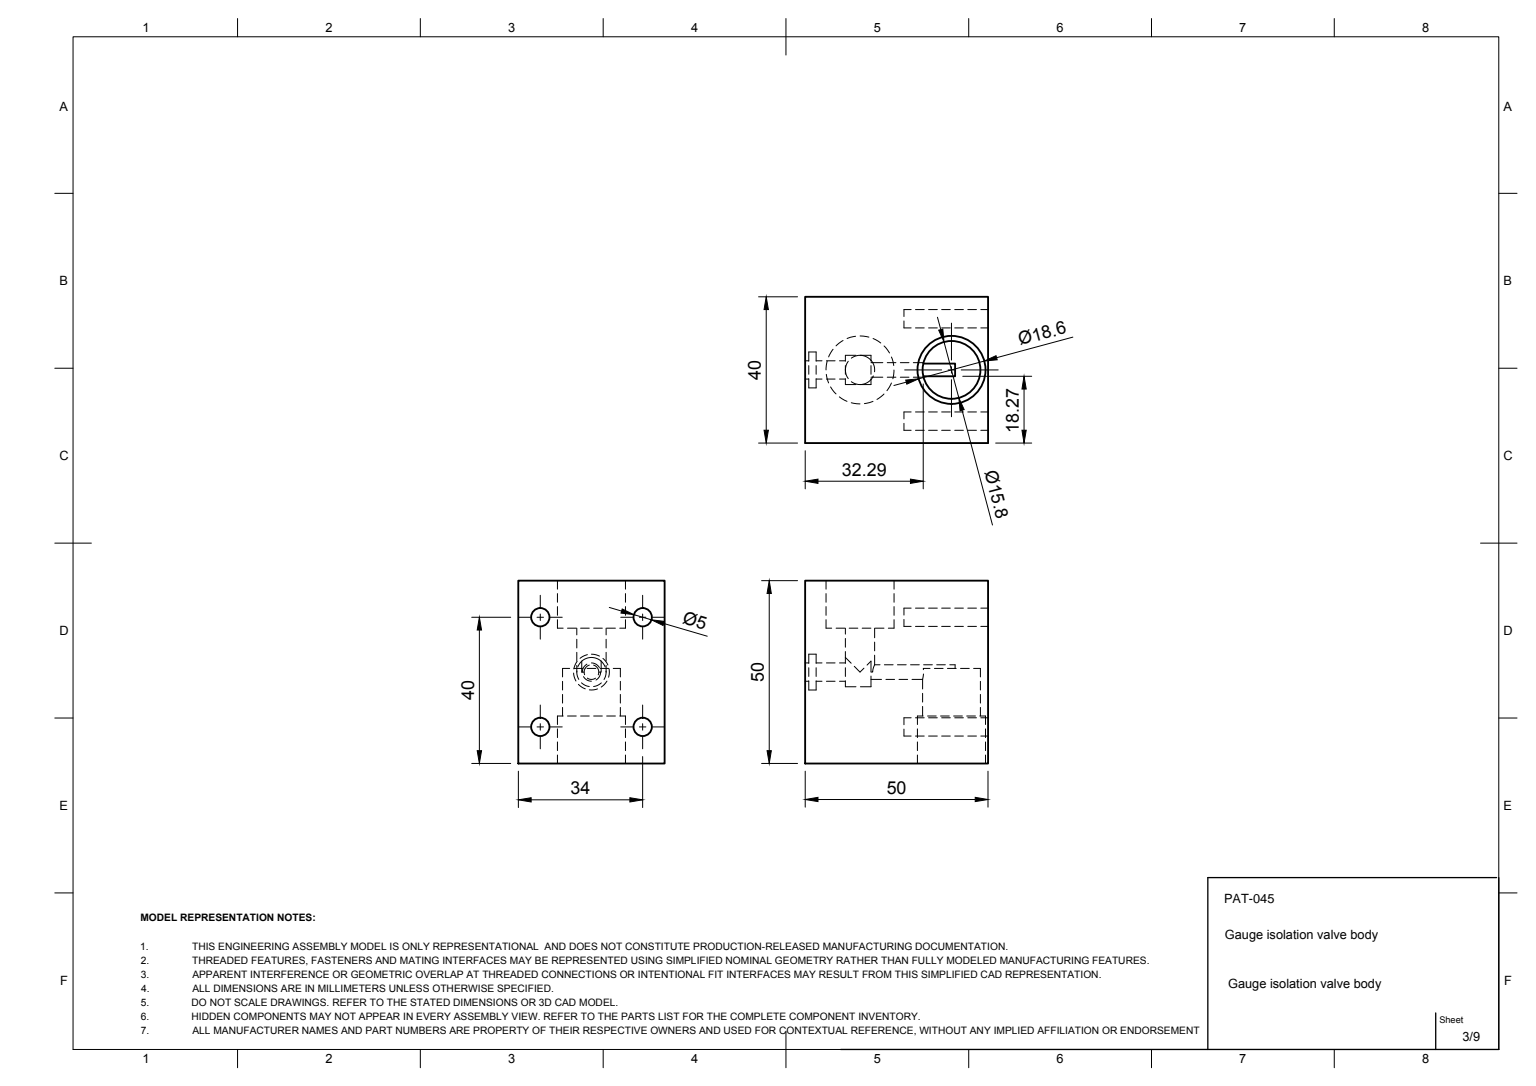
ISO-10303-21;
HEADER;
/* Generated by software containing ST-Developer
 * from STEP Tools, Inc. (www.steptools.com) 
 */

FILE_DESCRIPTION(
/* description */ ('Gauge isolation and snubber set'),
/* implementation_level */ '2;1');

FILE_NAME(
/* name */ 'Gauge isolation valve body.step',
/* time_stamp */ '2026-10-29T16:58:15-07:00',
/* author */ (''),
/* organization */ (''),
/* preprocessor_version */ 'ST-DEVELOPER v20.2',
/* originating_system */ 'Autodesk Translation Framework v15.17.0.0',
/* authorisation */ '');

FILE_SCHEMA (('AUTOMOTIVE_DESIGN { 1 0 10303 214 3 1 1 }'));
ENDSEC;

DATA;
#10=MECHANICAL_DESIGN_GEOMETRIC_PRESENTATION_REPRESENTATION('',(#92),#4043);
#76=SHAPE_REPRESENTATION_RELATIONSHIP('SRR','None',#4083,#84);
#84=ADVANCED_BREP_SHAPE_REPRESENTATION('',(#102),#4035);
#92=STYLED_ITEM('',(#4176),#102);
#102=MANIFOLD_SOLID_BREP('Body1',#2209);
#112=FACE_BOUND('',#379,.T.);
#113=FACE_BOUND('',#382,.T.);
#114=FACE_BOUND('',#384,.T.);
#115=FACE_BOUND('',#389,.T.);
#116=FACE_BOUND('',#397,.T.);
#117=FACE_BOUND('',#400,.T.);
#118=FACE_BOUND('',#403,.T.);
#119=FACE_BOUND('',#405,.T.);
#120=FACE_BOUND('',#407,.T.);
#121=FACE_BOUND('',#408,.T.);
#122=FACE_BOUND('',#409,.T.);
#123=FACE_BOUND('',#410,.T.);
#153=B_SPLINE_CURVE_WITH_KNOTS('',3,(#3286,#3287,#3288,#3289,#3290,#3291,
#3292,#3293,#3294,#3295,#3296,#3297,#3298,#3299,#3300,#3301,#3302,#3303),
 .UNSPECIFIED.,.F.,.F.,(4,2,2,2,2,2,2,2,4),(0.,0.0769830401762947,0.153966080352589,
0.230739261017803,0.307512441683016,0.384285622348229,0.461058803013443,
0.538041843189737,0.615024883366032),.UNSPECIFIED.);
#154=B_SPLINE_CURVE_WITH_KNOTS('',3,(#3360,#3361,#3362,#3363,#3364,#3365,
#3366,#3367,#3368,#3369,#3370,#3371,#3372,#3373,#3374),.UNSPECIFIED.,.F.,
 .F.,(4,2,2,2,3,2,4),(-0.302773934408822,-0.227086024595877,-0.151398114782933,
-0.0756990573914662,0.,0.0756990573914663,0.1003787904191),
 .UNSPECIFIED.);
#155=B_SPLINE_CURVE_WITH_KNOTS('',3,(#3377,#3378,#3379,#3380,#3381,#3382,
#3383,#3384,#3385,#3386,#3387,#3388,#3389,#3390),.UNSPECIFIED.,.F.,.F.,
(4,2,2,2,2,2,4),(-0.705926659236745,-0.681246926209111,-0.605547868817645,
-0.529848811426178,-0.454149754034712,-0.378461844221767,-0.302773934408822),
 .UNSPECIFIED.);
#164=PLANE('',#2319);
#165=PLANE('',#2323);
#166=PLANE('',#2327);
#167=PLANE('',#2331);
#168=PLANE('',#2332);
#169=PLANE('',#2339);
#170=PLANE('',#2343);
#171=PLANE('',#2347);
#172=PLANE('',#2349);
#173=PLANE('',#2358);
#174=PLANE('',#2359);
#175=PLANE('',#2362);
#176=PLANE('',#2365);
#177=PLANE('',#2372);
#178=PLANE('',#2373);
#179=PLANE('',#2374);
#180=PLANE('',#2375);
#181=PLANE('',#2376);
#182=PLANE('',#2377);
#183=PLANE('',#2378);
#241=FACE_OUTER_BOUND('',#365,.T.);
#242=FACE_OUTER_BOUND('',#366,.T.);
#243=FACE_OUTER_BOUND('',#367,.T.);
#244=FACE_OUTER_BOUND('',#368,.T.);
#245=FACE_OUTER_BOUND('',#369,.T.);
#246=FACE_OUTER_BOUND('',#370,.T.);
#247=FACE_OUTER_BOUND('',#371,.T.);
#248=FACE_OUTER_BOUND('',#372,.T.);
#249=FACE_OUTER_BOUND('',#373,.T.);
#250=FACE_OUTER_BOUND('',#374,.T.);
#251=FACE_OUTER_BOUND('',#375,.T.);
#252=FACE_OUTER_BOUND('',#376,.T.);
#253=FACE_OUTER_BOUND('',#377,.T.);
#254=FACE_OUTER_BOUND('',#378,.T.);
#255=FACE_OUTER_BOUND('',#380,.T.);
#256=FACE_OUTER_BOUND('',#381,.T.);
#257=FACE_OUTER_BOUND('',#383,.T.);
#258=FACE_OUTER_BOUND('',#385,.T.);
#259=FACE_OUTER_BOUND('',#386,.T.);
#260=FACE_OUTER_BOUND('',#387,.T.);
#261=FACE_OUTER_BOUND('',#388,.T.);
#262=FACE_OUTER_BOUND('',#390,.T.);
#263=FACE_OUTER_BOUND('',#391,.T.);
#264=FACE_OUTER_BOUND('',#392,.T.);
#265=FACE_OUTER_BOUND('',#393,.T.);
#266=FACE_OUTER_BOUND('',#394,.T.);
#267=FACE_OUTER_BOUND('',#395,.T.);
#268=FACE_OUTER_BOUND('',#396,.T.);
#269=FACE_OUTER_BOUND('',#398,.T.);
#270=FACE_OUTER_BOUND('',#399,.T.);
#271=FACE_OUTER_BOUND('',#401,.T.);
#272=FACE_OUTER_BOUND('',#402,.T.);
#273=FACE_OUTER_BOUND('',#404,.T.);
#274=FACE_OUTER_BOUND('',#406,.T.);
#365=EDGE_LOOP('',(#1461,#1462,#1463,#1464,#1465));
#366=EDGE_LOOP('',(#1466,#1467,#1468,#1469));
#367=EDGE_LOOP('',(#1470));
#368=EDGE_LOOP('',(#1471,#1472,#1473,#1474));
#369=EDGE_LOOP('',(#1475));
#370=EDGE_LOOP('',(#1476,#1477,#1478,#1479));
#371=EDGE_LOOP('',(#1480));
#372=EDGE_LOOP('',(#1481,#1482,#1483,#1484));
#373=EDGE_LOOP('',(#1485));
#374=EDGE_LOOP('',(#1486,#1487,#1488));
#375=EDGE_LOOP('',(#1489,#1490,#1491,#1492,#1493,#1494,#1495,#1496,#1497,
#1498,#1499,#1500));
#376=EDGE_LOOP('',(#1501,#1502,#1503));
#377=EDGE_LOOP('',(#1504,#1505,#1506,#1507));
#378=EDGE_LOOP('',(#1508));
#379=EDGE_LOOP('',(#1509));
#380=EDGE_LOOP('',(#1510,#1511,#1512,#1513));
#381=EDGE_LOOP('',(#1514));
#382=EDGE_LOOP('',(#1515));
#383=EDGE_LOOP('',(#1516));
#384=EDGE_LOOP('',(#1517));
#385=EDGE_LOOP('',(#1518,#1519,#1520,#1521));
#386=EDGE_LOOP('',(#1522,#1523,#1524,#1525));
#387=EDGE_LOOP('',(#1526,#1527,#1528,#1529,#1530));
#388=EDGE_LOOP('',(#1531,#1532));
#389=EDGE_LOOP('',(#1533));
#390=EDGE_LOOP('',(#1534,#1535,#1536,#1537,#1538,#1539,#1540,#1541));
#391=EDGE_LOOP('',(#1542,#1543));
#392=EDGE_LOOP('',(#1544,#1545,#1546,#1547,#1548,#1549,#1550,#1551,#1552,
#1553,#1554,#1555));
#393=EDGE_LOOP('',(#1556,#1557,#1558,#1559));
#394=EDGE_LOOP('',(#1560,#1561,#1562,#1563,#1564,#1565));
#395=EDGE_LOOP('',(#1566,#1567,#1568,#1569));
#396=EDGE_LOOP('',(#1570));
#397=EDGE_LOOP('',(#1571));
#398=EDGE_LOOP('',(#1572,#1573,#1574,#1575));
#399=EDGE_LOOP('',(#1576,#1577,#1578,#1579));
#400=EDGE_LOOP('',(#1580));
#401=EDGE_LOOP('',(#1581,#1582,#1583,#1584));
#402=EDGE_LOOP('',(#1585,#1586,#1587,#1588));
#403=EDGE_LOOP('',(#1589));
#404=EDGE_LOOP('',(#1590,#1591,#1592,#1593));
#405=EDGE_LOOP('',(#1594));
#406=EDGE_LOOP('',(#1595,#1596,#1597,#1598));
#407=EDGE_LOOP('',(#1599));
#408=EDGE_LOOP('',(#1600));
#409=EDGE_LOOP('',(#1601));
#410=EDGE_LOOP('',(#1602));
#530=ELLIPSE('',#2313,0.565685424949238,0.4);
#531=ELLIPSE('',#2314,0.565685424949238,0.4);
#532=ELLIPSE('',#2336,0.565685424949238,0.4);
#533=ELLIPSE('',#2337,0.565685424949238,0.4);
#534=CIRCLE('',#2312,0.4);
#535=CIRCLE('',#2315,0.4);
#536=CIRCLE('',#2317,0.25);
#537=CIRCLE('',#2318,0.25);
#538=CIRCLE('',#2321,0.25);
#539=CIRCLE('',#2322,0.25);
#540=CIRCLE('',#2325,0.25);
#541=CIRCLE('',#2326,0.25);
#542=CIRCLE('',#2329,0.25);
#543=CIRCLE('',#2330,0.25);
#544=CIRCLE('',#2333,0.4);
#545=CIRCLE('',#2335,0.4);
#546=CIRCLE('',#2338,0.4);
#547=CIRCLE('',#2341,0.93);
#548=CIRCLE('',#2342,0.93);
#549=CIRCLE('',#2345,0.49);
#550=CIRCLE('',#2346,0.49);
#551=CIRCLE('',#2348,0.25);
#552=CIRCLE('',#2350,0.25);
#553=CIRCLE('',#2352,0.25);
#554=CIRCLE('',#2354,0.25);
#555=CIRCLE('',#2356,0.4);
#556=CIRCLE('',#2357,0.4);
#557=CIRCLE('',#2360,0.2);
#558=CIRCLE('',#2361,0.2);
#559=CIRCLE('',#2363,0.2);
#560=CIRCLE('',#2366,0.79);
#561=CIRCLE('',#2368,0.79);
#562=CIRCLE('',#2370,0.93);
#563=CIRCLE('',#2371,0.93);
#634=LINE('',#3238,#805);
#635=LINE('',#3250,#806);
#636=LINE('',#3257,#807);
#637=LINE('',#3264,#808);
#638=LINE('',#3271,#809);
#639=LINE('',#3277,#810);
#640=LINE('',#3280,#811);
#641=LINE('',#3283,#812);
#642=LINE('',#3305,#813);
#643=LINE('',#3310,#814);
#644=LINE('',#3314,#815);
#645=LINE('',#3315,#816);
#646=LINE('',#3320,#817);
#647=LINE('',#3327,#818);
#648=LINE('',#3338,#819);
#649=LINE('',#3341,#820);
#650=LINE('',#3354,#821);
#651=LINE('',#3358,#822);
#652=LINE('',#3375,#823);
#653=LINE('',#3391,#824);
#654=LINE('',#3397,#825);
#655=LINE('',#3402,#826);
#656=LINE('',#3408,#827);
#657=LINE('',#3410,#828);
#658=LINE('',#3412,#829);
#659=LINE('',#3413,#830);
#660=LINE('',#3416,#831);
#661=LINE('',#3418,#832);
#662=LINE('',#3419,#833);
#663=LINE('',#3422,#834);
#664=LINE('',#3424,#835);
#665=LINE('',#3425,#836);
#666=LINE('',#3427,#837);
#667=LINE('',#3428,#838);
#805=VECTOR('',#2567,0.4);
#806=VECTOR('',#2580,0.25);
#807=VECTOR('',#2589,0.25);
#808=VECTOR('',#2598,0.25);
#809=VECTOR('',#2607,0.25);
#810=VECTOR('',#2614,1.);
#811=VECTOR('',#2617,1.);
#812=VECTOR('',#2620,1.);
#813=VECTOR('',#2623,1.);
#814=VECTOR('',#2628,0.4);
#815=VECTOR('',#2633,1.);
#816=VECTOR('',#2634,1.);
#817=VECTOR('',#2639,0.93);
#818=VECTOR('',#2648,0.49);
#819=VECTOR('',#2663,0.25);
#820=VECTOR('',#2666,0.25);
#821=VECTOR('',#2685,1.);
#822=VECTOR('',#2690,1.);
#823=VECTOR('',#2691,0.2);
#824=VECTOR('',#2692,1.);
#825=VECTOR('',#2701,0.79);
#826=VECTOR('',#2706,0.93);
#827=VECTOR('',#2713,1.);
#828=VECTOR('',#2714,1.);
#829=VECTOR('',#2715,1.);
#830=VECTOR('',#2716,1.);
#831=VECTOR('',#2719,1.);
#832=VECTOR('',#2720,1.);
#833=VECTOR('',#2721,1.);
#834=VECTOR('',#2724,1.);
#835=VECTOR('',#2725,1.);
#836=VECTOR('',#2726,1.);
#837=VECTOR('',#2729,1.);
#838=VECTOR('',#2730,1.);
#976=VERTEX_POINT('',#3236);
#977=VERTEX_POINT('',#3237);
#978=VERTEX_POINT('',#3239);
#979=VERTEX_POINT('',#3241);
#980=VERTEX_POINT('',#3243);
#981=VERTEX_POINT('',#3247);
#982=VERTEX_POINT('',#3249);
#983=VERTEX_POINT('',#3254);
#984=VERTEX_POINT('',#3256);
#985=VERTEX_POINT('',#3261);
#986=VERTEX_POINT('',#3263);
#987=VERTEX_POINT('',#3268);
#988=VERTEX_POINT('',#3270);
#989=VERTEX_POINT('',#3275);
#990=VERTEX_POINT('',#3276);
#991=VERTEX_POINT('',#3278);
#992=VERTEX_POINT('',#3282);
#993=VERTEX_POINT('',#3284);
#994=VERTEX_POINT('',#3304);
#995=VERTEX_POINT('',#3306);
#996=VERTEX_POINT('',#3309);
#997=VERTEX_POINT('',#3313);
#998=VERTEX_POINT('',#3317);
#999=VERTEX_POINT('',#3319);
#1000=VERTEX_POINT('',#3324);
#1001=VERTEX_POINT('',#3326);
#1002=VERTEX_POINT('',#3330);
#1003=VERTEX_POINT('',#3333);
#1004=VERTEX_POINT('',#3336);
#1005=VERTEX_POINT('',#3340);
#1006=VERTEX_POINT('',#3348);
#1007=VERTEX_POINT('',#3352);
#1008=VERTEX_POINT('',#3353);
#1009=VERTEX_POINT('',#3357);
#1010=VERTEX_POINT('',#3359);
#1011=VERTEX_POINT('',#3376);
#1012=VERTEX_POINT('',#3395);
#1013=VERTEX_POINT('',#3399);
#1014=VERTEX_POINT('',#3401);
#1015=VERTEX_POINT('',#3406);
#1016=VERTEX_POINT('',#3407);
#1017=VERTEX_POINT('',#3409);
#1018=VERTEX_POINT('',#3411);
#1019=VERTEX_POINT('',#3415);
#1020=VERTEX_POINT('',#3417);
#1021=VERTEX_POINT('',#3421);
#1022=VERTEX_POINT('',#3423);
#1169=EDGE_CURVE('',#976,#977,#634,.T.);
#1170=EDGE_CURVE('',#978,#976,#534,.T.);
#1171=EDGE_CURVE('',#978,#979,#530,.T.);
#1172=EDGE_CURVE('',#979,#980,#531,.T.);
#1173=EDGE_CURVE('',#980,#977,#535,.T.);
#1174=EDGE_CURVE('',#981,#981,#536,.T.);
#1175=EDGE_CURVE('',#981,#982,#635,.T.);
#1176=EDGE_CURVE('',#982,#982,#537,.T.);
#1177=EDGE_CURVE('',#983,#983,#538,.T.);
#1178=EDGE_CURVE('',#983,#984,#636,.T.);
#1179=EDGE_CURVE('',#984,#984,#539,.T.);
#1180=EDGE_CURVE('',#985,#985,#540,.T.);
#1181=EDGE_CURVE('',#985,#986,#637,.T.);
#1182=EDGE_CURVE('',#986,#986,#541,.T.);
#1183=EDGE_CURVE('',#987,#987,#542,.T.);
#1184=EDGE_CURVE('',#987,#988,#638,.T.);
#1185=EDGE_CURVE('',#988,#988,#543,.T.);
#1186=EDGE_CURVE('',#989,#990,#639,.T.);
#1187=EDGE_CURVE('',#989,#991,#544,.T.);
#1188=EDGE_CURVE('',#990,#991,#640,.T.);
#1189=EDGE_CURVE('',#992,#978,#641,.T.);
#1190=EDGE_CURVE('',#993,#992,#545,.T.);
#1191=EDGE_CURVE('',#991,#993,#153,.T.);
#1192=EDGE_CURVE('',#994,#989,#642,.T.);
#1193=EDGE_CURVE('',#995,#994,#532,.T.);
#1194=EDGE_CURVE('',#980,#995,#533,.T.);
#1195=EDGE_CURVE('',#980,#996,#643,.T.);
#1196=EDGE_CURVE('',#996,#996,#546,.T.);
#1197=EDGE_CURVE('',#997,#992,#644,.T.);
#1198=EDGE_CURVE('',#993,#997,#645,.T.);
#1199=EDGE_CURVE('',#998,#998,#547,.T.);
#1200=EDGE_CURVE('',#998,#999,#646,.T.);
#1201=EDGE_CURVE('',#999,#999,#548,.T.);
#1202=EDGE_CURVE('',#1000,#1000,#549,.T.);
#1203=EDGE_CURVE('',#1000,#1001,#647,.T.);
#1204=EDGE_CURVE('',#1001,#1001,#550,.T.);
#1205=EDGE_CURVE('',#1002,#1002,#551,.T.);
#1206=EDGE_CURVE('',#1003,#1003,#552,.T.);
#1207=EDGE_CURVE('',#1004,#1004,#553,.T.);
#1208=EDGE_CURVE('',#1004,#1003,#648,.T.);
#1209=EDGE_CURVE('',#1002,#1005,#649,.T.);
#1210=EDGE_CURVE('',#1005,#1005,#554,.T.);
#1211=EDGE_CURVE('',#977,#980,#555,.T.);
#1212=EDGE_CURVE('',#976,#994,#556,.T.);
#1213=EDGE_CURVE('',#1006,#990,#557,.T.);
#1214=EDGE_CURVE('',#997,#1006,#558,.T.);
#1215=EDGE_CURVE('',#1007,#1008,#650,.T.);
#1216=EDGE_CURVE('',#1007,#1008,#559,.T.);
#1217=EDGE_CURVE('',#1009,#1007,#651,.T.);
#1218=EDGE_CURVE('',#1010,#1009,#154,.T.);
#1219=EDGE_CURVE('',#1010,#1006,#652,.T.);
#1220=EDGE_CURVE('',#1011,#1010,#155,.T.);
#1221=EDGE_CURVE('',#1008,#1011,#653,.T.);
#1222=EDGE_CURVE('',#1009,#1011,#560,.T.);
#1223=EDGE_CURVE('',#1012,#1012,#561,.T.);
#1224=EDGE_CURVE('',#1012,#1010,#654,.T.);
#1225=EDGE_CURVE('',#1013,#1013,#562,.T.);
#1226=EDGE_CURVE('',#1013,#1014,#655,.T.);
#1227=EDGE_CURVE('',#1014,#1014,#563,.T.);
#1228=EDGE_CURVE('',#1015,#1016,#656,.T.);
#1229=EDGE_CURVE('',#1016,#1017,#657,.T.);
#1230=EDGE_CURVE('',#1018,#1017,#658,.T.);
#1231=EDGE_CURVE('',#1015,#1018,#659,.T.);
#1232=EDGE_CURVE('',#1019,#1015,#660,.T.);
#1233=EDGE_CURVE('',#1020,#1018,#661,.T.);
#1234=EDGE_CURVE('',#1019,#1020,#662,.T.);
#1235=EDGE_CURVE('',#1021,#1019,#663,.T.);
#1236=EDGE_CURVE('',#1022,#1020,#664,.T.);
#1237=EDGE_CURVE('',#1021,#1022,#665,.T.);
#1238=EDGE_CURVE('',#1016,#1021,#666,.T.);
#1239=EDGE_CURVE('',#1017,#1022,#667,.T.);
#1461=ORIENTED_EDGE('',*,*,#1169,.F.);
#1462=ORIENTED_EDGE('',*,*,#1170,.F.);
#1463=ORIENTED_EDGE('',*,*,#1171,.T.);
#1464=ORIENTED_EDGE('',*,*,#1172,.T.);
#1465=ORIENTED_EDGE('',*,*,#1173,.T.);
#1466=ORIENTED_EDGE('',*,*,#1174,.F.);
#1467=ORIENTED_EDGE('',*,*,#1175,.T.);
#1468=ORIENTED_EDGE('',*,*,#1176,.T.);
#1469=ORIENTED_EDGE('',*,*,#1175,.F.);
#1470=ORIENTED_EDGE('',*,*,#1176,.F.);
#1471=ORIENTED_EDGE('',*,*,#1177,.F.);
#1472=ORIENTED_EDGE('',*,*,#1178,.T.);
#1473=ORIENTED_EDGE('',*,*,#1179,.T.);
#1474=ORIENTED_EDGE('',*,*,#1178,.F.);
#1475=ORIENTED_EDGE('',*,*,#1179,.F.);
#1476=ORIENTED_EDGE('',*,*,#1180,.F.);
#1477=ORIENTED_EDGE('',*,*,#1181,.T.);
#1478=ORIENTED_EDGE('',*,*,#1182,.T.);
#1479=ORIENTED_EDGE('',*,*,#1181,.F.);
#1480=ORIENTED_EDGE('',*,*,#1182,.F.);
#1481=ORIENTED_EDGE('',*,*,#1183,.F.);
#1482=ORIENTED_EDGE('',*,*,#1184,.T.);
#1483=ORIENTED_EDGE('',*,*,#1185,.T.);
#1484=ORIENTED_EDGE('',*,*,#1184,.F.);
#1485=ORIENTED_EDGE('',*,*,#1185,.F.);
#1486=ORIENTED_EDGE('',*,*,#1186,.F.);
#1487=ORIENTED_EDGE('',*,*,#1187,.T.);
#1488=ORIENTED_EDGE('',*,*,#1188,.F.);
#1489=ORIENTED_EDGE('',*,*,#1189,.F.);
#1490=ORIENTED_EDGE('',*,*,#1190,.F.);
#1491=ORIENTED_EDGE('',*,*,#1191,.F.);
#1492=ORIENTED_EDGE('',*,*,#1187,.F.);
#1493=ORIENTED_EDGE('',*,*,#1192,.F.);
#1494=ORIENTED_EDGE('',*,*,#1193,.F.);
#1495=ORIENTED_EDGE('',*,*,#1194,.F.);
#1496=ORIENTED_EDGE('',*,*,#1195,.T.);
#1497=ORIENTED_EDGE('',*,*,#1196,.F.);
#1498=ORIENTED_EDGE('',*,*,#1195,.F.);
#1499=ORIENTED_EDGE('',*,*,#1172,.F.);
#1500=ORIENTED_EDGE('',*,*,#1171,.F.);
#1501=ORIENTED_EDGE('',*,*,#1197,.F.);
#1502=ORIENTED_EDGE('',*,*,#1198,.F.);
#1503=ORIENTED_EDGE('',*,*,#1190,.T.);
#1504=ORIENTED_EDGE('',*,*,#1199,.F.);
#1505=ORIENTED_EDGE('',*,*,#1200,.T.);
#1506=ORIENTED_EDGE('',*,*,#1201,.F.);
#1507=ORIENTED_EDGE('',*,*,#1200,.F.);
#1508=ORIENTED_EDGE('',*,*,#1199,.T.);
#1509=ORIENTED_EDGE('',*,*,#1196,.T.);
#1510=ORIENTED_EDGE('',*,*,#1202,.F.);
#1511=ORIENTED_EDGE('',*,*,#1203,.T.);
#1512=ORIENTED_EDGE('',*,*,#1204,.T.);
#1513=ORIENTED_EDGE('',*,*,#1203,.F.);
#1514=ORIENTED_EDGE('',*,*,#1204,.F.);
#1515=ORIENTED_EDGE('',*,*,#1205,.F.);
#1516=ORIENTED_EDGE('',*,*,#1202,.T.);
#1517=ORIENTED_EDGE('',*,*,#1206,.F.);
#1518=ORIENTED_EDGE('',*,*,#1207,.F.);
#1519=ORIENTED_EDGE('',*,*,#1208,.T.);
#1520=ORIENTED_EDGE('',*,*,#1206,.T.);
#1521=ORIENTED_EDGE('',*,*,#1208,.F.);
#1522=ORIENTED_EDGE('',*,*,#1205,.T.);
#1523=ORIENTED_EDGE('',*,*,#1209,.T.);
#1524=ORIENTED_EDGE('',*,*,#1210,.F.);
#1525=ORIENTED_EDGE('',*,*,#1209,.F.);
#1526=ORIENTED_EDGE('',*,*,#1169,.T.);
#1527=ORIENTED_EDGE('',*,*,#1211,.T.);
#1528=ORIENTED_EDGE('',*,*,#1194,.T.);
#1529=ORIENTED_EDGE('',*,*,#1193,.T.);
#1530=ORIENTED_EDGE('',*,*,#1212,.F.);
#1531=ORIENTED_EDGE('',*,*,#1173,.F.);
#1532=ORIENTED_EDGE('',*,*,#1211,.F.);
#1533=ORIENTED_EDGE('',*,*,#1207,.T.);
#1534=ORIENTED_EDGE('',*,*,#1189,.T.);
#1535=ORIENTED_EDGE('',*,*,#1170,.T.);
#1536=ORIENTED_EDGE('',*,*,#1212,.T.);
#1537=ORIENTED_EDGE('',*,*,#1192,.T.);
#1538=ORIENTED_EDGE('',*,*,#1186,.T.);
#1539=ORIENTED_EDGE('',*,*,#1213,.F.);
#1540=ORIENTED_EDGE('',*,*,#1214,.F.);
#1541=ORIENTED_EDGE('',*,*,#1197,.T.);
#1542=ORIENTED_EDGE('',*,*,#1215,.F.);
#1543=ORIENTED_EDGE('',*,*,#1216,.T.);
#1544=ORIENTED_EDGE('',*,*,#1217,.F.);
#1545=ORIENTED_EDGE('',*,*,#1218,.F.);
#1546=ORIENTED_EDGE('',*,*,#1219,.T.);
#1547=ORIENTED_EDGE('',*,*,#1213,.T.);
#1548=ORIENTED_EDGE('',*,*,#1188,.T.);
#1549=ORIENTED_EDGE('',*,*,#1191,.T.);
#1550=ORIENTED_EDGE('',*,*,#1198,.T.);
#1551=ORIENTED_EDGE('',*,*,#1214,.T.);
#1552=ORIENTED_EDGE('',*,*,#1219,.F.);
#1553=ORIENTED_EDGE('',*,*,#1220,.F.);
#1554=ORIENTED_EDGE('',*,*,#1221,.F.);
#1555=ORIENTED_EDGE('',*,*,#1216,.F.);
#1556=ORIENTED_EDGE('',*,*,#1217,.T.);
#1557=ORIENTED_EDGE('',*,*,#1215,.T.);
#1558=ORIENTED_EDGE('',*,*,#1221,.T.);
#1559=ORIENTED_EDGE('',*,*,#1222,.F.);
#1560=ORIENTED_EDGE('',*,*,#1223,.F.);
#1561=ORIENTED_EDGE('',*,*,#1224,.T.);
#1562=ORIENTED_EDGE('',*,*,#1218,.T.);
#1563=ORIENTED_EDGE('',*,*,#1222,.T.);
#1564=ORIENTED_EDGE('',*,*,#1220,.T.);
#1565=ORIENTED_EDGE('',*,*,#1224,.F.);
#1566=ORIENTED_EDGE('',*,*,#1225,.F.);
#1567=ORIENTED_EDGE('',*,*,#1226,.T.);
#1568=ORIENTED_EDGE('',*,*,#1227,.T.);
#1569=ORIENTED_EDGE('',*,*,#1226,.F.);
#1570=ORIENTED_EDGE('',*,*,#1227,.F.);
#1571=ORIENTED_EDGE('',*,*,#1223,.T.);
#1572=ORIENTED_EDGE('',*,*,#1228,.T.);
#1573=ORIENTED_EDGE('',*,*,#1229,.T.);
#1574=ORIENTED_EDGE('',*,*,#1230,.F.);
#1575=ORIENTED_EDGE('',*,*,#1231,.F.);
#1576=ORIENTED_EDGE('',*,*,#1232,.T.);
#1577=ORIENTED_EDGE('',*,*,#1231,.T.);
#1578=ORIENTED_EDGE('',*,*,#1233,.F.);
#1579=ORIENTED_EDGE('',*,*,#1234,.F.);
#1580=ORIENTED_EDGE('',*,*,#1201,.T.);
#1581=ORIENTED_EDGE('',*,*,#1235,.T.);
#1582=ORIENTED_EDGE('',*,*,#1234,.T.);
#1583=ORIENTED_EDGE('',*,*,#1236,.F.);
#1584=ORIENTED_EDGE('',*,*,#1237,.F.);
#1585=ORIENTED_EDGE('',*,*,#1238,.T.);
#1586=ORIENTED_EDGE('',*,*,#1237,.T.);
#1587=ORIENTED_EDGE('',*,*,#1239,.F.);
#1588=ORIENTED_EDGE('',*,*,#1229,.F.);
#1589=ORIENTED_EDGE('',*,*,#1225,.T.);
#1590=ORIENTED_EDGE('',*,*,#1239,.T.);
#1591=ORIENTED_EDGE('',*,*,#1236,.T.);
#1592=ORIENTED_EDGE('',*,*,#1233,.T.);
#1593=ORIENTED_EDGE('',*,*,#1230,.T.);
#1594=ORIENTED_EDGE('',*,*,#1210,.T.);
#1595=ORIENTED_EDGE('',*,*,#1238,.F.);
#1596=ORIENTED_EDGE('',*,*,#1228,.F.);
#1597=ORIENTED_EDGE('',*,*,#1232,.F.);
#1598=ORIENTED_EDGE('',*,*,#1235,.F.);
#1599=ORIENTED_EDGE('',*,*,#1174,.T.);
#1600=ORIENTED_EDGE('',*,*,#1177,.T.);
#1601=ORIENTED_EDGE('',*,*,#1180,.T.);
#1602=ORIENTED_EDGE('',*,*,#1183,.T.);
#2045=CYLINDRICAL_SURFACE('',#2311,0.4);
#2046=CYLINDRICAL_SURFACE('',#2316,0.25);
#2047=CYLINDRICAL_SURFACE('',#2320,0.25);
#2048=CYLINDRICAL_SURFACE('',#2324,0.25);
#2049=CYLINDRICAL_SURFACE('',#2328,0.25);
#2050=CYLINDRICAL_SURFACE('',#2334,0.4);
#2051=CYLINDRICAL_SURFACE('',#2340,0.93);
#2052=CYLINDRICAL_SURFACE('',#2344,0.49);
#2053=CYLINDRICAL_SURFACE('',#2351,0.25);
#2054=CYLINDRICAL_SURFACE('',#2353,0.25);
#2055=CYLINDRICAL_SURFACE('',#2355,0.4);
#2056=CYLINDRICAL_SURFACE('',#2364,0.2);
#2057=CYLINDRICAL_SURFACE('',#2367,0.79);
#2058=CYLINDRICAL_SURFACE('',#2369,0.93);
#2085=ADVANCED_FACE('',(#241),#2045,.F.);
#2086=ADVANCED_FACE('',(#242),#2046,.F.);
#2087=ADVANCED_FACE('',(#243),#164,.F.);
#2088=ADVANCED_FACE('',(#244),#2047,.F.);
#2089=ADVANCED_FACE('',(#245),#165,.F.);
#2090=ADVANCED_FACE('',(#246),#2048,.F.);
#2091=ADVANCED_FACE('',(#247),#166,.F.);
#2092=ADVANCED_FACE('',(#248),#2049,.F.);
#2093=ADVANCED_FACE('',(#249),#167,.F.);
#2094=ADVANCED_FACE('',(#250),#168,.T.);
#2095=ADVANCED_FACE('',(#251),#2050,.F.);
#2096=ADVANCED_FACE('',(#252),#169,.T.);
#2097=ADVANCED_FACE('',(#253),#2051,.F.);
#2098=ADVANCED_FACE('',(#254,#112),#170,.T.);
#2099=ADVANCED_FACE('',(#255),#2052,.F.);
#2100=ADVANCED_FACE('',(#256,#113),#171,.F.);
#2101=ADVANCED_FACE('',(#257,#114),#172,.T.);
#2102=ADVANCED_FACE('',(#258),#2053,.F.);
#2103=ADVANCED_FACE('',(#259),#2054,.F.);
#2104=ADVANCED_FACE('',(#260),#2055,.F.);
#2105=ADVANCED_FACE('',(#261,#115),#173,.F.);
#2106=ADVANCED_FACE('',(#262),#174,.T.);
#2107=ADVANCED_FACE('',(#263),#175,.T.);
#2108=ADVANCED_FACE('',(#264),#2056,.F.);
#2109=ADVANCED_FACE('',(#265),#176,.F.);
#2110=ADVANCED_FACE('',(#266),#2057,.F.);
#2111=ADVANCED_FACE('',(#267),#2058,.F.);
#2112=ADVANCED_FACE('',(#268,#116),#177,.F.);
#2113=ADVANCED_FACE('',(#269),#178,.T.);
#2114=ADVANCED_FACE('',(#270,#117),#179,.T.);
#2115=ADVANCED_FACE('',(#271),#180,.T.);
#2116=ADVANCED_FACE('',(#272,#118),#181,.T.);
#2117=ADVANCED_FACE('',(#273,#119),#182,.T.);
#2118=ADVANCED_FACE('',(#274,#120,#121,#122,#123),#183,.F.);
#2209=CLOSED_SHELL('',(#2085,#2086,#2087,#2088,#2089,#2090,#2091,#2092,
#2093,#2094,#2095,#2096,#2097,#2098,#2099,#2100,#2101,#2102,#2103,#2104,
#2105,#2106,#2107,#2108,#2109,#2110,#2111,#2112,#2113,#2114,#2115,#2116,
#2117,#2118));
#2310=AXIS2_PLACEMENT_3D('',#3234,#2563,#2564);
#2311=AXIS2_PLACEMENT_3D('',#3235,#2565,#2566);
#2312=AXIS2_PLACEMENT_3D('',#3240,#2568,#2569);
#2313=AXIS2_PLACEMENT_3D('',#3242,#2570,#2571);
#2314=AXIS2_PLACEMENT_3D('',#3244,#2572,#2573);
#2315=AXIS2_PLACEMENT_3D('',#3245,#2574,#2575);
#2316=AXIS2_PLACEMENT_3D('',#3246,#2576,#2577);
#2317=AXIS2_PLACEMENT_3D('',#3248,#2578,#2579);
#2318=AXIS2_PLACEMENT_3D('',#3251,#2581,#2582);
#2319=AXIS2_PLACEMENT_3D('',#3252,#2583,#2584);
#2320=AXIS2_PLACEMENT_3D('',#3253,#2585,#2586);
#2321=AXIS2_PLACEMENT_3D('',#3255,#2587,#2588);
#2322=AXIS2_PLACEMENT_3D('',#3258,#2590,#2591);
#2323=AXIS2_PLACEMENT_3D('',#3259,#2592,#2593);
#2324=AXIS2_PLACEMENT_3D('',#3260,#2594,#2595);
#2325=AXIS2_PLACEMENT_3D('',#3262,#2596,#2597);
#2326=AXIS2_PLACEMENT_3D('',#3265,#2599,#2600);
#2327=AXIS2_PLACEMENT_3D('',#3266,#2601,#2602);
#2328=AXIS2_PLACEMENT_3D('',#3267,#2603,#2604);
#2329=AXIS2_PLACEMENT_3D('',#3269,#2605,#2606);
#2330=AXIS2_PLACEMENT_3D('',#3272,#2608,#2609);
#2331=AXIS2_PLACEMENT_3D('',#3273,#2610,#2611);
#2332=AXIS2_PLACEMENT_3D('',#3274,#2612,#2613);
#2333=AXIS2_PLACEMENT_3D('',#3279,#2615,#2616);
#2334=AXIS2_PLACEMENT_3D('',#3281,#2618,#2619);
#2335=AXIS2_PLACEMENT_3D('',#3285,#2621,#2622);
#2336=AXIS2_PLACEMENT_3D('',#3307,#2624,#2625);
#2337=AXIS2_PLACEMENT_3D('',#3308,#2626,#2627);
#2338=AXIS2_PLACEMENT_3D('',#3311,#2629,#2630);
#2339=AXIS2_PLACEMENT_3D('',#3312,#2631,#2632);
#2340=AXIS2_PLACEMENT_3D('',#3316,#2635,#2636);
#2341=AXIS2_PLACEMENT_3D('',#3318,#2637,#2638);
#2342=AXIS2_PLACEMENT_3D('',#3321,#2640,#2641);
#2343=AXIS2_PLACEMENT_3D('',#3322,#2642,#2643);
#2344=AXIS2_PLACEMENT_3D('',#3323,#2644,#2645);
#2345=AXIS2_PLACEMENT_3D('',#3325,#2646,#2647);
#2346=AXIS2_PLACEMENT_3D('',#3328,#2649,#2650);
#2347=AXIS2_PLACEMENT_3D('',#3329,#2651,#2652);
#2348=AXIS2_PLACEMENT_3D('',#3331,#2653,#2654);
#2349=AXIS2_PLACEMENT_3D('',#3332,#2655,#2656);
#2350=AXIS2_PLACEMENT_3D('',#3334,#2657,#2658);
#2351=AXIS2_PLACEMENT_3D('',#3335,#2659,#2660);
#2352=AXIS2_PLACEMENT_3D('',#3337,#2661,#2662);
#2353=AXIS2_PLACEMENT_3D('',#3339,#2664,#2665);
#2354=AXIS2_PLACEMENT_3D('',#3342,#2667,#2668);
#2355=AXIS2_PLACEMENT_3D('',#3343,#2669,#2670);
#2356=AXIS2_PLACEMENT_3D('',#3344,#2671,#2672);
#2357=AXIS2_PLACEMENT_3D('',#3345,#2673,#2674);
#2358=AXIS2_PLACEMENT_3D('',#3346,#2675,#2676);
#2359=AXIS2_PLACEMENT_3D('',#3347,#2677,#2678);
#2360=AXIS2_PLACEMENT_3D('',#3349,#2679,#2680);
#2361=AXIS2_PLACEMENT_3D('',#3350,#2681,#2682);
#2362=AXIS2_PLACEMENT_3D('',#3351,#2683,#2684);
#2363=AXIS2_PLACEMENT_3D('',#3355,#2686,#2687);
#2364=AXIS2_PLACEMENT_3D('',#3356,#2688,#2689);
#2365=AXIS2_PLACEMENT_3D('',#3392,#2693,#2694);
#2366=AXIS2_PLACEMENT_3D('',#3393,#2695,#2696);
#2367=AXIS2_PLACEMENT_3D('',#3394,#2697,#2698);
#2368=AXIS2_PLACEMENT_3D('',#3396,#2699,#2700);
#2369=AXIS2_PLACEMENT_3D('',#3398,#2702,#2703);
#2370=AXIS2_PLACEMENT_3D('',#3400,#2704,#2705);
#2371=AXIS2_PLACEMENT_3D('',#3403,#2707,#2708);
#2372=AXIS2_PLACEMENT_3D('',#3404,#2709,#2710);
#2373=AXIS2_PLACEMENT_3D('',#3405,#2711,#2712);
#2374=AXIS2_PLACEMENT_3D('',#3414,#2717,#2718);
#2375=AXIS2_PLACEMENT_3D('',#3420,#2722,#2723);
#2376=AXIS2_PLACEMENT_3D('',#3426,#2727,#2728);
#2377=AXIS2_PLACEMENT_3D('',#3429,#2731,#2732);
#2378=AXIS2_PLACEMENT_3D('',#3430,#2733,#2734);
#2563=DIRECTION('axis',(0.,0.,1.));
#2564=DIRECTION('refdir',(1.,0.,0.));
#2565=DIRECTION('center_axis',(0.,0.,1.));
#2566=DIRECTION('ref_axis',(1.,0.,0.));
#2567=DIRECTION('',(0.,0.,1.));
#2568=DIRECTION('center_axis',(0.,0.,1.));
#2569=DIRECTION('ref_axis',(1.,0.,0.));
#2570=DIRECTION('center_axis',(0.707106781186548,0.,0.707106781186547));
#2571=DIRECTION('ref_axis',(0.707106781186547,0.,-0.707106781186548));
#2572=DIRECTION('center_axis',(0.707106781186548,0.,-0.707106781186547));
#2573=DIRECTION('ref_axis',(-0.707106781186547,0.,-0.707106781186548));
#2574=DIRECTION('center_axis',(0.,0.,1.));
#2575=DIRECTION('ref_axis',(1.,0.,0.));
#2576=DIRECTION('center_axis',(0.,0.,1.));
#2577=DIRECTION('ref_axis',(1.,0.,0.));
#2578=DIRECTION('center_axis',(0.,0.,1.));
#2579=DIRECTION('ref_axis',(1.,0.,0.));
#2580=DIRECTION('',(0.,0.,1.));
#2581=DIRECTION('center_axis',(0.,0.,1.));
#2582=DIRECTION('ref_axis',(1.,0.,0.));
#2583=DIRECTION('center_axis',(0.,0.,1.));
#2584=DIRECTION('ref_axis',(1.,0.,0.));
#2585=DIRECTION('center_axis',(0.,0.,1.));
#2586=DIRECTION('ref_axis',(1.,0.,0.));
#2587=DIRECTION('center_axis',(0.,0.,1.));
#2588=DIRECTION('ref_axis',(1.,0.,0.));
#2589=DIRECTION('',(0.,0.,1.));
#2590=DIRECTION('center_axis',(0.,0.,1.));
#2591=DIRECTION('ref_axis',(1.,0.,0.));
#2592=DIRECTION('center_axis',(0.,0.,1.));
#2593=DIRECTION('ref_axis',(1.,0.,0.));
#2594=DIRECTION('center_axis',(0.,0.,1.));
#2595=DIRECTION('ref_axis',(1.,0.,0.));
#2596=DIRECTION('center_axis',(0.,0.,1.));
#2597=DIRECTION('ref_axis',(1.,0.,0.));
#2598=DIRECTION('',(0.,0.,1.));
#2599=DIRECTION('center_axis',(0.,0.,1.));
#2600=DIRECTION('ref_axis',(1.,0.,0.));
#2601=DIRECTION('center_axis',(0.,0.,1.));
#2602=DIRECTION('ref_axis',(1.,0.,0.));
#2603=DIRECTION('center_axis',(0.,0.,1.));
#2604=DIRECTION('ref_axis',(1.,0.,0.));
#2605=DIRECTION('center_axis',(0.,0.,1.));
#2606=DIRECTION('ref_axis',(1.,0.,0.));
#2607=DIRECTION('',(0.,0.,1.));
#2608=DIRECTION('center_axis',(0.,0.,1.));
#2609=DIRECTION('ref_axis',(1.,0.,0.));
#2610=DIRECTION('center_axis',(0.,0.,1.));
#2611=DIRECTION('ref_axis',(1.,0.,0.));
#2612=DIRECTION('center_axis',(1.,0.,0.));
#2613=DIRECTION('ref_axis',(0.,0.,-1.));
#2614=DIRECTION('',(0.,1.,0.));
#2615=DIRECTION('center_axis',(1.,0.,0.));
#2616=DIRECTION('ref_axis',(0.,0.,-1.));
#2617=DIRECTION('',(0.,0.,-1.));
#2618=DIRECTION('center_axis',(1.,0.,0.));
#2619=DIRECTION('ref_axis',(0.,0.,-1.));
#2620=DIRECTION('',(1.,0.,0.));
#2621=DIRECTION('center_axis',(1.,0.,0.));
#2622=DIRECTION('ref_axis',(0.,0.,-1.));
#2623=DIRECTION('',(-1.,0.,0.));
#2624=DIRECTION('center_axis',(0.707106781186548,0.,0.707106781186547));
#2625=DIRECTION('ref_axis',(0.707106781186547,0.,-0.707106781186548));
#2626=DIRECTION('center_axis',(0.707106781186548,0.,-0.707106781186547));
#2627=DIRECTION('ref_axis',(-0.707106781186547,0.,-0.707106781186548));
#2628=DIRECTION('',(1.,0.,0.));
#2629=DIRECTION('center_axis',(-1.,0.,0.));
#2630=DIRECTION('ref_axis',(0.,0.,-1.));
#2631=DIRECTION('center_axis',(1.,0.,0.));
#2632=DIRECTION('ref_axis',(0.,0.,-1.));
#2633=DIRECTION('',(0.,1.,0.));
#2634=DIRECTION('',(0.,0.,1.));
#2635=DIRECTION('center_axis',(1.,0.,0.));
#2636=DIRECTION('ref_axis',(0.,0.,-1.));
#2637=DIRECTION('center_axis',(1.,0.,0.));
#2638=DIRECTION('ref_axis',(0.,0.,-1.));
#2639=DIRECTION('',(1.,0.,0.));
#2640=DIRECTION('center_axis',(-1.,0.,0.));
#2641=DIRECTION('ref_axis',(0.,0.,-1.));
#2642=DIRECTION('center_axis',(1.,0.,0.));
#2643=DIRECTION('ref_axis',(0.,0.,-1.));
#2644=DIRECTION('center_axis',(0.,0.,1.));
#2645=DIRECTION('ref_axis',(1.,0.,0.));
#2646=DIRECTION('center_axis',(0.,0.,1.));
#2647=DIRECTION('ref_axis',(1.,0.,0.));
#2648=DIRECTION('',(0.,0.,1.));
#2649=DIRECTION('center_axis',(0.,0.,1.));
#2650=DIRECTION('ref_axis',(1.,0.,0.));
#2651=DIRECTION('center_axis',(0.,0.,1.));
#2652=DIRECTION('ref_axis',(1.,0.,0.));
#2653=DIRECTION('center_axis',(0.,0.,-1.));
#2654=DIRECTION('ref_axis',(1.,0.,0.));
#2655=DIRECTION('center_axis',(0.,0.,1.));
#2656=DIRECTION('ref_axis',(1.,0.,0.));
#2657=DIRECTION('center_axis',(0.,0.,1.));
#2658=DIRECTION('ref_axis',(1.,0.,0.));
#2659=DIRECTION('center_axis',(0.,0.,1.));
#2660=DIRECTION('ref_axis',(1.,0.,0.));
#2661=DIRECTION('center_axis',(0.,0.,1.));
#2662=DIRECTION('ref_axis',(1.,0.,0.));
#2663=DIRECTION('',(0.,0.,1.));
#2664=DIRECTION('center_axis',(0.,0.,1.));
#2665=DIRECTION('ref_axis',(1.,0.,0.));
#2666=DIRECTION('',(0.,0.,1.));
#2667=DIRECTION('center_axis',(0.,0.,-1.));
#2668=DIRECTION('ref_axis',(1.,0.,0.));
#2669=DIRECTION('center_axis',(0.,0.,1.));
#2670=DIRECTION('ref_axis',(1.,0.,0.));
#2671=DIRECTION('center_axis',(0.,0.,1.));
#2672=DIRECTION('ref_axis',(1.,0.,0.));
#2673=DIRECTION('center_axis',(0.,0.,1.));
#2674=DIRECTION('ref_axis',(1.,0.,0.));
#2675=DIRECTION('center_axis',(0.,0.,1.));
#2676=DIRECTION('ref_axis',(1.,0.,0.));
#2677=DIRECTION('center_axis',(0.,0.,1.));
#2678=DIRECTION('ref_axis',(1.,0.,0.));
#2679=DIRECTION('center_axis',(0.,0.,1.));
#2680=DIRECTION('ref_axis',(1.,0.,0.));
#2681=DIRECTION('center_axis',(0.,0.,1.));
#2682=DIRECTION('ref_axis',(1.,0.,0.));
#2683=DIRECTION('center_axis',(0.,0.,1.));
#2684=DIRECTION('ref_axis',(1.,0.,0.));
#2685=DIRECTION('',(0.,1.,0.));
#2686=DIRECTION('center_axis',(0.,0.,1.));
#2687=DIRECTION('ref_axis',(1.,0.,0.));
#2688=DIRECTION('center_axis',(0.,0.,1.));
#2689=DIRECTION('ref_axis',(1.,0.,0.));
#2690=DIRECTION('',(0.,0.,-1.));
#2691=DIRECTION('',(0.,0.,1.));
#2692=DIRECTION('',(0.,0.,1.));
#2693=DIRECTION('center_axis',(1.,0.,0.));
#2694=DIRECTION('ref_axis',(0.,0.,-1.));
#2695=DIRECTION('center_axis',(1.,0.,0.));
#2696=DIRECTION('ref_axis',(0.,0.,-1.));
#2697=DIRECTION('center_axis',(1.,0.,0.));
#2698=DIRECTION('ref_axis',(0.,0.,-1.));
#2699=DIRECTION('center_axis',(1.,0.,0.));
#2700=DIRECTION('ref_axis',(0.,0.,-1.));
#2701=DIRECTION('',(1.,0.,0.));
#2702=DIRECTION('center_axis',(1.,0.,0.));
#2703=DIRECTION('ref_axis',(0.,0.,-1.));
#2704=DIRECTION('center_axis',(1.,0.,0.));
#2705=DIRECTION('ref_axis',(0.,0.,-1.));
#2706=DIRECTION('',(1.,0.,0.));
#2707=DIRECTION('center_axis',(1.,0.,0.));
#2708=DIRECTION('ref_axis',(0.,0.,-1.));
#2709=DIRECTION('center_axis',(1.,0.,0.));
#2710=DIRECTION('ref_axis',(0.,0.,-1.));
#2711=DIRECTION('center_axis',(0.,1.,0.));
#2712=DIRECTION('ref_axis',(-1.,0.,0.));
#2713=DIRECTION('',(-1.,0.,0.));
#2714=DIRECTION('',(0.,0.,1.));
#2715=DIRECTION('',(-1.,0.,0.));
#2716=DIRECTION('',(0.,0.,1.));
#2717=DIRECTION('center_axis',(1.,0.,0.));
#2718=DIRECTION('ref_axis',(0.,1.,0.));
#2719=DIRECTION('',(0.,1.,0.));
#2720=DIRECTION('',(0.,1.,0.));
#2721=DIRECTION('',(0.,0.,1.));
#2722=DIRECTION('center_axis',(0.,-1.,0.));
#2723=DIRECTION('ref_axis',(1.,0.,0.));
#2724=DIRECTION('',(1.,0.,0.));
#2725=DIRECTION('',(1.,0.,0.));
#2726=DIRECTION('',(0.,0.,1.));
#2727=DIRECTION('center_axis',(-1.,0.,0.));
#2728=DIRECTION('ref_axis',(0.,-1.,0.));
#2729=DIRECTION('',(0.,-1.,0.));
#2730=DIRECTION('',(0.,-1.,0.));
#2731=DIRECTION('center_axis',(0.,0.,1.));
#2732=DIRECTION('ref_axis',(1.,0.,0.));
#2733=DIRECTION('center_axis',(0.,0.,1.));
#2734=DIRECTION('ref_axis',(1.,0.,0.));
#3234=CARTESIAN_POINT('',(0.,0.,0.));
#3235=CARTESIAN_POINT('Origin',(0.,0.,8.2));
#3236=CARTESIAN_POINT('',(-0.4,-4.89858719658941E-17,8.2));
#3237=CARTESIAN_POINT('',(-0.4,-4.89858719658941E-17,8.9));
#3238=CARTESIAN_POINT('',(-0.4,-4.89858719658941E-17,8.2));
#3239=CARTESIAN_POINT('',(0.299999999999998,0.264575131106461,8.2));
#3240=CARTESIAN_POINT('Origin',(0.,0.,8.2));
#3241=CARTESIAN_POINT('',(0.,0.4,8.5));
#3242=CARTESIAN_POINT('Origin',(0.,0.,8.5));
#3243=CARTESIAN_POINT('',(0.4,0.,8.9));
#3244=CARTESIAN_POINT('Origin',(0.,0.,8.5));
#3245=CARTESIAN_POINT('Origin',(0.,0.,8.9));
#3246=CARTESIAN_POINT('Origin',(1.5,1.4,4.9));
#3247=CARTESIAN_POINT('',(1.25,1.4,5.));
#3248=CARTESIAN_POINT('Origin',(1.5,1.4,5.));
#3249=CARTESIAN_POINT('',(1.25,1.4,7.3));
#3250=CARTESIAN_POINT('',(1.25,1.4,4.9));
#3251=CARTESIAN_POINT('Origin',(1.5,1.4,7.3));
#3252=CARTESIAN_POINT('Origin',(1.5,1.4,7.3));
#3253=CARTESIAN_POINT('Origin',(1.5,-1.4,4.9));
#3254=CARTESIAN_POINT('',(1.25,-1.4,5.));
#3255=CARTESIAN_POINT('Origin',(1.5,-1.4,5.));
#3256=CARTESIAN_POINT('',(1.25,-1.4,7.3));
#3257=CARTESIAN_POINT('',(1.25,-1.4,4.9));
#3258=CARTESIAN_POINT('Origin',(1.5,-1.4,7.3));
#3259=CARTESIAN_POINT('Origin',(1.5,-1.4,7.3));
#3260=CARTESIAN_POINT('Origin',(-1.5,1.4,4.9));
#3261=CARTESIAN_POINT('',(-1.75,1.4,5.));
#3262=CARTESIAN_POINT('Origin',(-1.5,1.4,5.));
#3263=CARTESIAN_POINT('',(-1.75,1.4,7.3));
#3264=CARTESIAN_POINT('',(-1.75,1.4,4.9));
#3265=CARTESIAN_POINT('Origin',(-1.5,1.4,7.3));
#3266=CARTESIAN_POINT('Origin',(-1.5,1.4,7.3));
#3267=CARTESIAN_POINT('Origin',(-1.5,-1.4,4.9));
#3268=CARTESIAN_POINT('',(-1.75,-1.4,5.));
#3269=CARTESIAN_POINT('Origin',(-1.5,-1.4,5.));
#3270=CARTESIAN_POINT('',(-1.75,-1.4,7.3));
#3271=CARTESIAN_POINT('',(-1.75,-1.4,4.9));
#3272=CARTESIAN_POINT('Origin',(-1.5,-1.4,7.3));
#3273=CARTESIAN_POINT('Origin',(-1.5,-1.4,7.3));
#3274=CARTESIAN_POINT('Origin',(0.,0.,8.5));
#3275=CARTESIAN_POINT('',(0.,-0.264575131106461,8.2));
#3276=CARTESIAN_POINT('',(0.,-0.2,8.2));
#3277=CARTESIAN_POINT('',(0.,0.,8.2));
#3278=CARTESIAN_POINT('',(0.,-0.2,8.15358983848622));
#3279=CARTESIAN_POINT('Origin',(0.,0.,8.5));
#3280=CARTESIAN_POINT('',(0.,-0.2,5.9));
#3281=CARTESIAN_POINT('Origin',(0.,0.,8.5));
#3282=CARTESIAN_POINT('',(0.,0.264575131106461,8.2));
#3283=CARTESIAN_POINT('',(0.,0.264575131106461,8.2));
#3284=CARTESIAN_POINT('',(0.,0.2,8.15358983848622));
#3285=CARTESIAN_POINT('Origin',(0.,0.,8.5));
#3286=CARTESIAN_POINT('Ctrl Pts',(-6.93889390390723E-18,-0.2,8.15358983848622));
#3287=CARTESIAN_POINT('Ctrl Pts',(0.0256610133920982,-0.2,8.15358983848622));
#3288=CARTESIAN_POINT('Ctrl Pts',(0.0526277202526568,-0.194777116895352,
8.15043491280941));
#3289=CARTESIAN_POINT('Ctrl Pts',(0.101716471901564,-0.174245741947245,
8.13976079750786));
#3290=CARTESIAN_POINT('Ctrl Pts',(0.123891546848412,-0.158951165626207,
8.13245990649023));
#3291=CARTESIAN_POINT('Ctrl Pts',(0.158903378513366,-0.123939333961253,
8.1192266779859));
#3292=CARTESIAN_POINT('Ctrl Pts',(0.174233015984916,-0.101748151622875,
8.1123470317921));
#3293=CARTESIAN_POINT('Ctrl Pts',(0.194792781173826,-0.0525890150977706,
8.10268160632987));
#3294=CARTESIAN_POINT('Ctrl Pts',(0.2,-0.0255910602217378,8.1));
#3295=CARTESIAN_POINT('Ctrl Pts',(0.2,0.0255910602217378,8.1));
#3296=CARTESIAN_POINT('Ctrl Pts',(0.194792781173826,0.0525890150977706,
8.10268160632987));
#3297=CARTESIAN_POINT('Ctrl Pts',(0.174233015984916,0.101748151622875,8.1123470317921));
#3298=CARTESIAN_POINT('Ctrl Pts',(0.158903378513366,0.123939333961253,8.1192266779859));
#3299=CARTESIAN_POINT('Ctrl Pts',(0.123891546848412,0.158951165626207,8.13245990649023));
#3300=CARTESIAN_POINT('Ctrl Pts',(0.101716471901564,0.174245741947245,8.13976079750786));
#3301=CARTESIAN_POINT('Ctrl Pts',(0.0526277202526568,0.194777116895352,
8.15043491280941));
#3302=CARTESIAN_POINT('Ctrl Pts',(0.0256610133920983,0.2,8.15358983848622));
#3303=CARTESIAN_POINT('Ctrl Pts',(2.08166817117217E-17,0.2,8.15358983848622));
#3304=CARTESIAN_POINT('',(0.299999999999998,-0.264575131106461,8.2));
#3305=CARTESIAN_POINT('',(0.,-0.264575131106461,8.2));
#3306=CARTESIAN_POINT('',(0.,-0.4,8.5));
#3307=CARTESIAN_POINT('Origin',(0.,0.,8.5));
#3308=CARTESIAN_POINT('Origin',(0.,0.,8.5));
#3309=CARTESIAN_POINT('',(1.2,4.89858719658942E-17,8.9));
#3310=CARTESIAN_POINT('',(0.,-4.89858719658942E-17,8.9));
#3311=CARTESIAN_POINT('Origin',(1.2,0.,8.5));
#3312=CARTESIAN_POINT('Origin',(0.,0.,8.5));
#3313=CARTESIAN_POINT('',(0.,0.2,8.2));
#3314=CARTESIAN_POINT('',(0.,0.,8.2));
#3315=CARTESIAN_POINT('',(0.,0.2,5.9));
#3316=CARTESIAN_POINT('Origin',(1.2,0.,8.5));
#3317=CARTESIAN_POINT('',(1.2,-1.13892152320704E-16,9.43));
#3318=CARTESIAN_POINT('Origin',(1.2,0.,8.5));
#3319=CARTESIAN_POINT('',(2.5,1.13892152320704E-16,9.43));
#3320=CARTESIAN_POINT('',(1.2,-1.13892152320704E-16,9.43));
#3321=CARTESIAN_POINT('Origin',(2.5,0.,8.5));
#3322=CARTESIAN_POINT('Origin',(1.2,0.,8.5));
#3323=CARTESIAN_POINT('Origin',(0.,0.,9.7));
#3324=CARTESIAN_POINT('',(-0.49,-6.00076931582203E-17,9.7));
#3325=CARTESIAN_POINT('Origin',(0.,0.,9.7));
#3326=CARTESIAN_POINT('',(-0.49,-6.00076931582203E-17,9.9));
#3327=CARTESIAN_POINT('',(-0.49,-6.00076931582203E-17,9.7));
#3328=CARTESIAN_POINT('Origin',(0.,0.,9.9));
#3329=CARTESIAN_POINT('Origin',(0.,0.,9.9));
#3330=CARTESIAN_POINT('',(-0.25,3.06161699786838E-17,9.9));
#3331=CARTESIAN_POINT('Origin',(0.,0.,9.9));
#3332=CARTESIAN_POINT('Origin',(0.,0.,9.7));
#3333=CARTESIAN_POINT('',(-0.25,-3.06161699786838E-17,9.7));
#3334=CARTESIAN_POINT('Origin',(0.,0.,9.7));
#3335=CARTESIAN_POINT('Origin',(0.,0.,8.8));
#3336=CARTESIAN_POINT('',(-0.25,-3.06161699786838E-17,8.9));
#3337=CARTESIAN_POINT('Origin',(0.,0.,8.9));
#3338=CARTESIAN_POINT('',(-0.25,-3.06161699786838E-17,8.8));
#3339=CARTESIAN_POINT('Origin',(0.,0.,8.8));
#3340=CARTESIAN_POINT('',(-0.25,3.06161699786838E-17,10.));
#3341=CARTESIAN_POINT('',(-0.25,-3.06161699786838E-17,8.8));
#3342=CARTESIAN_POINT('Origin',(0.,0.,10.));
#3343=CARTESIAN_POINT('Origin',(0.,0.,8.2));
#3344=CARTESIAN_POINT('Origin',(0.,0.,8.9));
#3345=CARTESIAN_POINT('Origin',(0.,0.,8.2));
#3346=CARTESIAN_POINT('Origin',(0.,0.,8.9));
#3347=CARTESIAN_POINT('Origin',(0.,0.,8.2));
#3348=CARTESIAN_POINT('',(-0.2,-2.44929359829471E-17,8.2));
#3349=CARTESIAN_POINT('Origin',(0.,0.,8.2));
#3350=CARTESIAN_POINT('Origin',(0.,0.,8.2));
#3351=CARTESIAN_POINT('Origin',(0.,0.,5.9));
#3352=CARTESIAN_POINT('',(0.1,-0.173205080756888,5.9));
#3353=CARTESIAN_POINT('',(0.1,0.173205080756888,5.9));
#3354=CARTESIAN_POINT('',(0.1,0.,5.9));
#3355=CARTESIAN_POINT('Origin',(0.,0.,5.9));
#3356=CARTESIAN_POINT('Origin',(0.,0.,5.9));
#3357=CARTESIAN_POINT('',(0.1,-0.173205080756888,6.77077882690172));
#3358=CARTESIAN_POINT('',(0.1,-0.173205080756888,5.9));
#3359=CARTESIAN_POINT('',(-0.2,-3.65325966551488E-17,6.79));
#3360=CARTESIAN_POINT('Ctrl Pts',(-0.2,-3.46944695195361E-17,6.79));
#3361=CARTESIAN_POINT('Ctrl Pts',(-0.2,-0.0252293032709816,6.79));
#3362=CARTESIAN_POINT('Ctrl Pts',(-0.194935517523083,-0.0520663682763995,
6.78867047644404));
#3363=CARTESIAN_POINT('Ctrl Pts',(-0.174490207856786,-0.101311053228714,
6.78386739800365));
#3364=CARTESIAN_POINT('Ctrl Pts',(-0.159115319800683,-0.123727392673936,
6.78045818190283));
#3365=CARTESIAN_POINT('Ctrl Pts',(-0.123724786645461,-0.159117925829158,
6.77401874806683));
#3366=CARTESIAN_POINT('Ctrl Pts',(-0.101309531057858,-0.174490782742294,
6.77056050717812));
#3367=CARTESIAN_POINT('Ctrl Pts',(-0.0520686947820295,-0.19493460869448,
6.76564419277622));
#3368=CARTESIAN_POINT('Ctrl Pts',(-0.0252330191304887,-0.2,6.76426435217142));
#3369=CARTESIAN_POINT('Ctrl Pts',(0.,-0.2,6.76426435217142));
#3370=CARTESIAN_POINT('Ctrl Pts',(0.0252330191304888,-0.2,6.76426435217142));
#3371=CARTESIAN_POINT('Ctrl Pts',(0.0520686947820297,-0.19493460869448,
6.76564419277622));
#3372=CARTESIAN_POINT('Ctrl Pts',(0.0847159677793139,-0.181380103583493,
6.76890376898488));
#3373=CARTESIAN_POINT('Ctrl Pts',(0.0925218917477068,-0.177522568569378,
6.7698086253353));
#3374=CARTESIAN_POINT('Ctrl Pts',(0.1,-0.173205080756888,6.77077882690173));
#3375=CARTESIAN_POINT('',(-0.2,-2.44929359829471E-17,5.9));
#3376=CARTESIAN_POINT('',(0.1,0.173205080756888,6.77077882690172));
#3377=CARTESIAN_POINT('Ctrl Pts',(0.1,0.173205080756888,6.77077882690173));
#3378=CARTESIAN_POINT('Ctrl Pts',(0.0925218917477067,0.177522568569378,
6.7698086253353));
#3379=CARTESIAN_POINT('Ctrl Pts',(0.0847159677793139,0.181380103583493,
6.76890376898488));
#3380=CARTESIAN_POINT('Ctrl Pts',(0.0520686947820296,0.19493460869448,6.76564419277622));
#3381=CARTESIAN_POINT('Ctrl Pts',(0.0252330191304888,0.2,6.76426435217142));
#3382=CARTESIAN_POINT('Ctrl Pts',(-0.0252330191304888,0.2,6.76426435217142));
#3383=CARTESIAN_POINT('Ctrl Pts',(-0.0520686947820297,0.19493460869448,
6.76564419277622));
#3384=CARTESIAN_POINT('Ctrl Pts',(-0.101309531057858,0.174490782742294,
6.77056050717812));
#3385=CARTESIAN_POINT('Ctrl Pts',(-0.123724786645461,0.159117925829158,
6.77401874806683));
#3386=CARTESIAN_POINT('Ctrl Pts',(-0.159115319800683,0.123727392673936,
6.78045818190283));
#3387=CARTESIAN_POINT('Ctrl Pts',(-0.174490207856786,0.101311053228714,
6.78386739800365));
#3388=CARTESIAN_POINT('Ctrl Pts',(-0.194935517523083,0.0520663682763994,
6.78867047644404));
#3389=CARTESIAN_POINT('Ctrl Pts',(-0.2,0.0252293032709816,6.79));
#3390=CARTESIAN_POINT('Ctrl Pts',(-0.2,-6.24500451351651E-17,6.79));
#3391=CARTESIAN_POINT('',(0.1,0.173205080756888,5.9));
#3392=CARTESIAN_POINT('Origin',(0.1,0.,6.));
#3393=CARTESIAN_POINT('Origin',(0.1,0.,6.));
#3394=CARTESIAN_POINT('Origin',(-1.3,0.,6.));
#3395=CARTESIAN_POINT('',(-1.2,-9.67470971326409E-17,6.79));
#3396=CARTESIAN_POINT('Origin',(-1.2,0.,6.));
#3397=CARTESIAN_POINT('',(-1.3,-9.67470971326409E-17,6.79));
#3398=CARTESIAN_POINT('Origin',(-2.6,0.,6.));
#3399=CARTESIAN_POINT('',(-2.5,-1.13892152320704E-16,6.93));
#3400=CARTESIAN_POINT('Origin',(-2.5,0.,6.));
#3401=CARTESIAN_POINT('',(-1.2,-1.13892152320704E-16,6.93));
#3402=CARTESIAN_POINT('',(-2.6,-1.13892152320704E-16,6.93));
#3403=CARTESIAN_POINT('Origin',(-1.2,0.,6.));
#3404=CARTESIAN_POINT('Origin',(-1.2,0.,6.));
#3405=CARTESIAN_POINT('Origin',(2.5,2.,5.));
#3406=CARTESIAN_POINT('',(2.5,2.,5.));
#3407=CARTESIAN_POINT('',(-2.5,2.,5.));
#3408=CARTESIAN_POINT('',(2.5,2.,5.));
#3409=CARTESIAN_POINT('',(-2.5,2.,10.));
#3410=CARTESIAN_POINT('',(-2.5,2.,5.));
#3411=CARTESIAN_POINT('',(2.5,2.,10.));
#3412=CARTESIAN_POINT('',(2.5,2.,10.));
#3413=CARTESIAN_POINT('',(2.5,2.,5.));
#3414=CARTESIAN_POINT('Origin',(2.5,-2.,5.));
#3415=CARTESIAN_POINT('',(2.5,-2.,5.));
#3416=CARTESIAN_POINT('',(2.5,-2.,5.));
#3417=CARTESIAN_POINT('',(2.5,-2.,10.));
#3418=CARTESIAN_POINT('',(2.5,-2.,10.));
#3419=CARTESIAN_POINT('',(2.5,-2.,5.));
#3420=CARTESIAN_POINT('Origin',(-2.5,-2.,5.));
#3421=CARTESIAN_POINT('',(-2.5,-2.,5.));
#3422=CARTESIAN_POINT('',(-2.5,-2.,5.));
#3423=CARTESIAN_POINT('',(-2.5,-2.,10.));
#3424=CARTESIAN_POINT('',(-2.5,-2.,10.));
#3425=CARTESIAN_POINT('',(-2.5,-2.,5.));
#3426=CARTESIAN_POINT('Origin',(-2.5,2.,5.));
#3427=CARTESIAN_POINT('',(-2.5,2.,5.));
#3428=CARTESIAN_POINT('',(-2.5,2.,10.));
#3429=CARTESIAN_POINT('Origin',(0.,0.,10.));
#3430=CARTESIAN_POINT('Origin',(0.,0.,5.));
#4024=UNCERTAINTY_MEASURE_WITH_UNIT(LENGTH_MEASURE(0.001),#4044,
'DISTANCE_ACCURACY_VALUE',
'Maximum model space distance between geometric entities at asserted c
onnectivities');
#4032=UNCERTAINTY_MEASURE_WITH_UNIT(LENGTH_MEASURE(0.001),#4044,
'DISTANCE_ACCURACY_VALUE',
'Maximum model space distance between geometric entities at asserted c
onnectivities');
#4035=(
GEOMETRIC_REPRESENTATION_CONTEXT(3)
GLOBAL_UNCERTAINTY_ASSIGNED_CONTEXT((#4024))
GLOBAL_UNIT_ASSIGNED_CONTEXT((#4044,#4046,#4047))
REPRESENTATION_CONTEXT('','3D')
);
#4043=(
GEOMETRIC_REPRESENTATION_CONTEXT(3)
GLOBAL_UNCERTAINTY_ASSIGNED_CONTEXT((#4032))
GLOBAL_UNIT_ASSIGNED_CONTEXT((#4044,#4046,#4047))
REPRESENTATION_CONTEXT('','3D')
);
#4044=(
LENGTH_UNIT()
NAMED_UNIT(*)
SI_UNIT(.CENTI.,.METRE.)
);
#4046=(
NAMED_UNIT(*)
PLANE_ANGLE_UNIT()
SI_UNIT($,.RADIAN.)
);
#4047=(
NAMED_UNIT(*)
SI_UNIT($,.STERADIAN.)
SOLID_ANGLE_UNIT()
);
#4050=SHAPE_DEFINITION_REPRESENTATION(#4060,#4083);
#4060=PRODUCT_DEFINITION_SHAPE('',$,#4094);
#4083=SHAPE_REPRESENTATION('',(#2310),#4035);
#4091=PRODUCT_DEFINITION_CONTEXT('part definition',#4123,'design');
#4094=PRODUCT_DEFINITION('Gauge isolation valve body',
'Gauge isolation valve body',#4104,#4091);
#4104=PRODUCT_DEFINITION_FORMATION('',$,#4127);
#4123=APPLICATION_CONTEXT(
'Core Data for Automotive Mechanical Design Process');
#4124=PRODUCT_CONTEXT('part definition',#4123,'mechanical');
#4127=PRODUCT('Gauge isolation valve body','Gauge isolation valve body',
'Gauge isolation valve body',(#4124));
#4170=COLOUR_RGB('Dark Blue',0.08,0.2,0.34);
#4171=FILL_AREA_STYLE_COLOUR('',#4170);
#4172=FILL_AREA_STYLE('',(#4171));
#4173=SURFACE_STYLE_FILL_AREA(#4172);
#4174=SURFACE_SIDE_STYLE('',(#4173));
#4175=SURFACE_STYLE_USAGE(.BOTH.,#4174);
#4176=PRESENTATION_STYLE_ASSIGNMENT((#4175));
ENDSEC;
END-ISO-10303-21;
